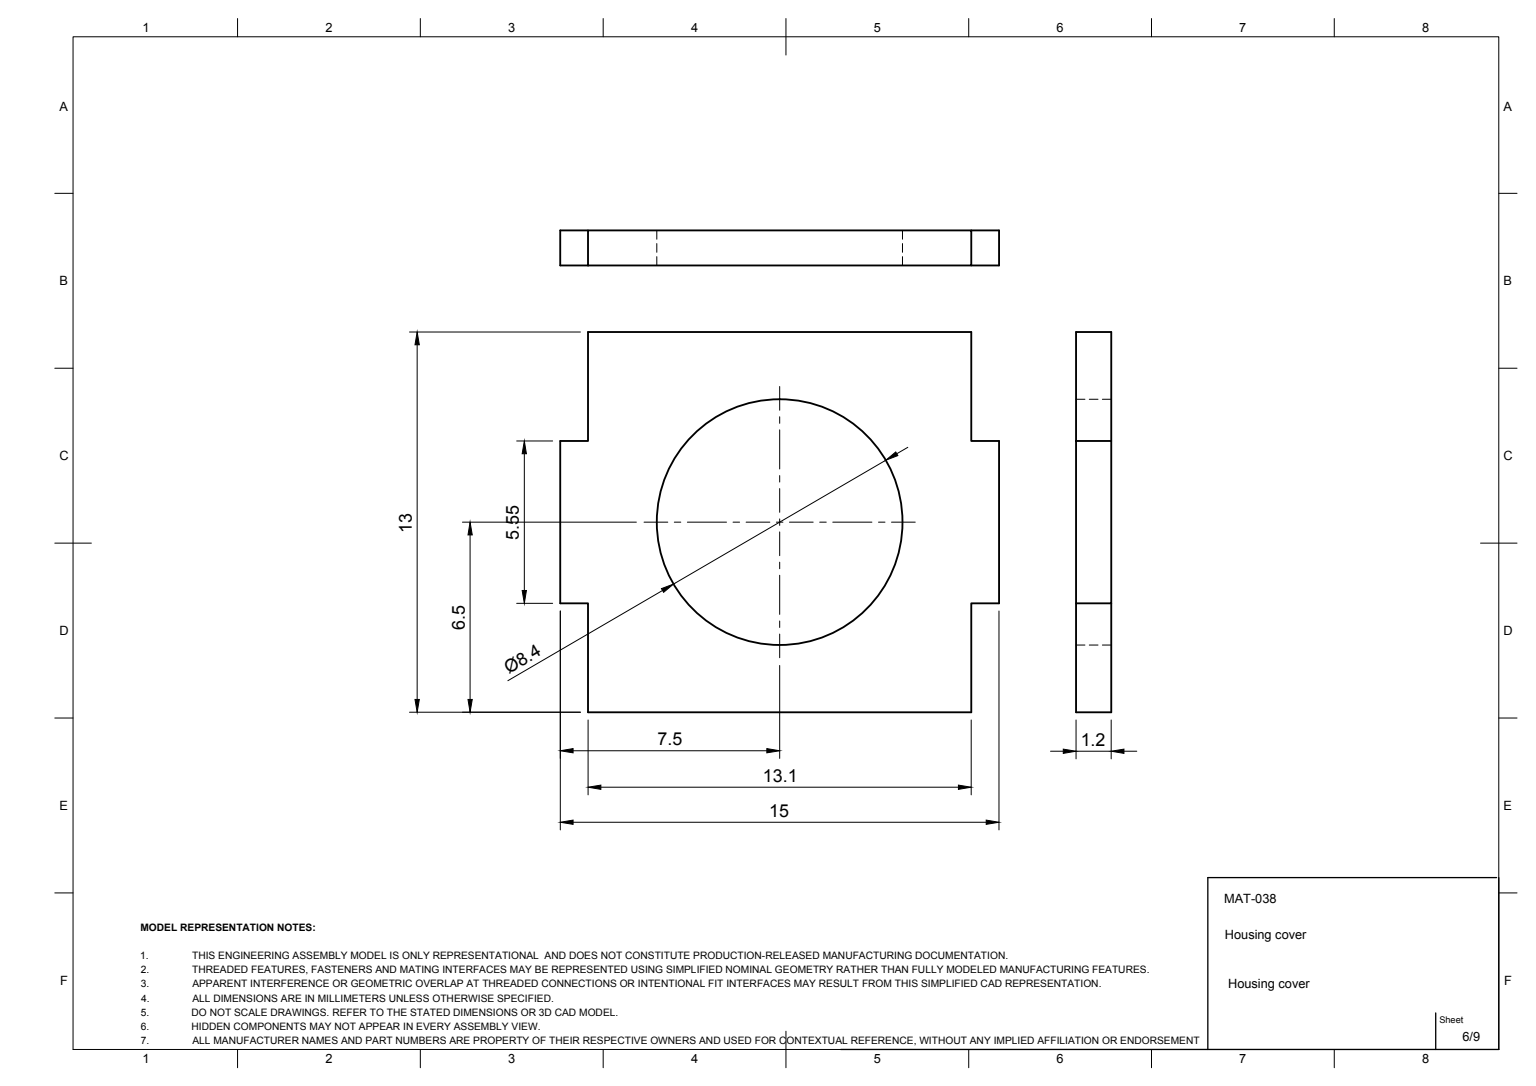
ISO-10303-21;
HEADER;
/* Generated by software containing ST-Developer
 * from STEP Tools, Inc. (www.steptools.com) 
 */

FILE_DESCRIPTION(
/* description */ ('STEP AP214'),
/* implementation_level */ '2;1');

FILE_NAME(
/* name */ 'Housing Cover.step',
/* time_stamp */ '2026-11-14T21:32:33-08:00',
/* author */ (''),
/* organization */ (''),
/* preprocessor_version */ 'ST-DEVELOPER v20.2',
/* originating_system */ 'Autodesk Translation Framework v15.17.0.0',
/* authorisation */ '');

FILE_SCHEMA (('AUTOMOTIVE_DESIGN { 1 0 10303 214 3 1 1 }'));
ENDSEC;

DATA;
#10=MECHANICAL_DESIGN_GEOMETRIC_PRESENTATION_REPRESENTATION('',(#180),#10551);
#162=SHAPE_REPRESENTATION_RELATIONSHIP('SRR','None',#10589,#171);
#171=ADVANCED_BREP_SHAPE_REPRESENTATION('',(#190),#10545);
#180=STYLED_ITEM('',(#10640),#190);
#190=MANIFOLD_SOLID_BREP('Body1',#3429);
#210=FACE_BOUND('',#586,.T.);
#211=FACE_BOUND('',#588,.T.);
#257=PLANE('',#3637);
#258=PLANE('',#3638);
#259=PLANE('',#3639);
#260=PLANE('',#3640);
#261=PLANE('',#3641);
#262=PLANE('',#3642);
#263=PLANE('',#3643);
#264=PLANE('',#3644);
#265=PLANE('',#3645);
#266=PLANE('',#3646);
#267=PLANE('',#3647);
#268=PLANE('',#3648);
#269=PLANE('',#3649);
#270=PLANE('',#3650);
#347=FACE_OUTER_BOUND('',#580,.T.);
#348=FACE_OUTER_BOUND('',#581,.T.);
#349=FACE_OUTER_BOUND('',#582,.T.);
#350=FACE_OUTER_BOUND('',#583,.T.);
#351=FACE_OUTER_BOUND('',#584,.T.);
#352=FACE_OUTER_BOUND('',#585,.T.);
#353=FACE_OUTER_BOUND('',#587,.T.);
#354=FACE_OUTER_BOUND('',#589,.T.);
#355=FACE_OUTER_BOUND('',#590,.T.);
#356=FACE_OUTER_BOUND('',#591,.T.);
#357=FACE_OUTER_BOUND('',#592,.T.);
#358=FACE_OUTER_BOUND('',#593,.T.);
#359=FACE_OUTER_BOUND('',#594,.T.);
#360=FACE_OUTER_BOUND('',#595,.T.);
#361=FACE_OUTER_BOUND('',#596,.T.);
#580=EDGE_LOOP('',(#2452,#2453,#2454,#2455));
#581=EDGE_LOOP('',(#2456,#2457,#2458,#2459));
#582=EDGE_LOOP('',(#2460,#2461,#2462,#2463));
#583=EDGE_LOOP('',(#2464,#2465,#2466,#2467));
#584=EDGE_LOOP('',(#2468,#2469,#2470,#2471));
#585=EDGE_LOOP('',(#2472,#2473,#2474,#2475,#2476,#2477,#2478,#2479,#2480,
#2481,#2482,#2483));
#586=EDGE_LOOP('',(#2484));
#587=EDGE_LOOP('',(#2485,#2486,#2487,#2488,#2489,#2490,#2491,#2492,#2493,
#2494,#2495,#2496));
#588=EDGE_LOOP('',(#2497));
#589=EDGE_LOOP('',(#2498,#2499,#2500,#2501));
#590=EDGE_LOOP('',(#2502,#2503,#2504,#2505));
#591=EDGE_LOOP('',(#2506,#2507,#2508,#2509));
#592=EDGE_LOOP('',(#2510,#2511,#2512,#2513));
#593=EDGE_LOOP('',(#2514,#2515,#2516,#2517));
#594=EDGE_LOOP('',(#2518,#2519,#2520,#2521));
#595=EDGE_LOOP('',(#2522,#2523,#2524,#2525));
#596=EDGE_LOOP('',(#2526,#2527,#2528,#2529));
#853=LINE('',#5515,#1050);
#854=LINE('',#5520,#1051);
#855=LINE('',#5522,#1052);
#856=LINE('',#5524,#1053);
#857=LINE('',#5525,#1054);
#858=LINE('',#5529,#1055);
#859=LINE('',#5531,#1056);
#860=LINE('',#5533,#1057);
#861=LINE('',#5534,#1058);
#862=LINE('',#5538,#1059);
#863=LINE('',#5540,#1060);
#864=LINE('',#5542,#1061);
#865=LINE('',#5543,#1062);
#866=LINE('',#5547,#1063);
#867=LINE('',#5549,#1064);
#868=LINE('',#5551,#1065);
#869=LINE('',#5552,#1066);
#870=LINE('',#5555,#1067);
#871=LINE('',#5556,#1068);
#872=LINE('',#5558,#1069);
#873=LINE('',#5559,#1070);
#874=LINE('',#5561,#1071);
#875=LINE('',#5562,#1072);
#876=LINE('',#5564,#1073);
#877=LINE('',#5565,#1074);
#878=LINE('',#5568,#1075);
#879=LINE('',#5569,#1076);
#880=LINE('',#5571,#1077);
#881=LINE('',#5572,#1078);
#882=LINE('',#5574,#1079);
#883=LINE('',#5575,#1080);
#884=LINE('',#5577,#1081);
#885=LINE('',#5578,#1082);
#886=LINE('',#5580,#1083);
#887=LINE('',#5583,#1084);
#888=LINE('',#5586,#1085);
#889=LINE('',#5589,#1086);
#1050=VECTOR('',#4328,4.2);
#1051=VECTOR('',#4333,1000.);
#1052=VECTOR('',#4334,1000.);
#1053=VECTOR('',#4335,1000.);
#1054=VECTOR('',#4336,1000.);
#1055=VECTOR('',#4339,1000.);
#1056=VECTOR('',#4340,1000.);
#1057=VECTOR('',#4341,1000.);
#1058=VECTOR('',#4342,1000.);
#1059=VECTOR('',#4345,1000.);
#1060=VECTOR('',#4346,1000.);
#1061=VECTOR('',#4347,1000.);
#1062=VECTOR('',#4348,1000.);
#1063=VECTOR('',#4351,1000.);
#1064=VECTOR('',#4352,1000.);
#1065=VECTOR('',#4353,1000.);
#1066=VECTOR('',#4354,1000.);
#1067=VECTOR('',#4357,1000.);
#1068=VECTOR('',#4358,1000.);
#1069=VECTOR('',#4359,1000.);
#1070=VECTOR('',#4360,1000.);
#1071=VECTOR('',#4361,1000.);
#1072=VECTOR('',#4362,1000.);
#1073=VECTOR('',#4363,1000.);
#1074=VECTOR('',#4364,1000.);
#1075=VECTOR('',#4367,1000.);
#1076=VECTOR('',#4368,1000.);
#1077=VECTOR('',#4369,1000.);
#1078=VECTOR('',#4370,1000.);
#1079=VECTOR('',#4371,1000.);
#1080=VECTOR('',#4372,1000.);
#1081=VECTOR('',#4373,1000.);
#1082=VECTOR('',#4374,1000.);
#1083=VECTOR('',#4377,1000.);
#1084=VECTOR('',#4382,1000.);
#1085=VECTOR('',#4387,1000.);
#1086=VECTOR('',#4392,1000.);
#1195=CIRCLE('',#3635,4.2);
#1196=CIRCLE('',#3636,4.2);
#1509=VERTEX_POINT('',#5512);
#1510=VERTEX_POINT('',#5514);
#1511=VERTEX_POINT('',#5518);
#1512=VERTEX_POINT('',#5519);
#1513=VERTEX_POINT('',#5521);
#1514=VERTEX_POINT('',#5523);
#1515=VERTEX_POINT('',#5527);
#1516=VERTEX_POINT('',#5528);
#1517=VERTEX_POINT('',#5530);
#1518=VERTEX_POINT('',#5532);
#1519=VERTEX_POINT('',#5536);
#1520=VERTEX_POINT('',#5537);
#1521=VERTEX_POINT('',#5539);
#1522=VERTEX_POINT('',#5541);
#1523=VERTEX_POINT('',#5545);
#1524=VERTEX_POINT('',#5546);
#1525=VERTEX_POINT('',#5548);
#1526=VERTEX_POINT('',#5550);
#1527=VERTEX_POINT('',#5554);
#1528=VERTEX_POINT('',#5557);
#1529=VERTEX_POINT('',#5560);
#1530=VERTEX_POINT('',#5563);
#1531=VERTEX_POINT('',#5567);
#1532=VERTEX_POINT('',#5570);
#1533=VERTEX_POINT('',#5573);
#1534=VERTEX_POINT('',#5576);
#1839=EDGE_CURVE('',#1509,#1509,#1195,.T.);
#1840=EDGE_CURVE('',#1509,#1510,#853,.T.);
#1841=EDGE_CURVE('',#1510,#1510,#1196,.T.);
#1842=EDGE_CURVE('',#1511,#1512,#854,.T.);
#1843=EDGE_CURVE('',#1513,#1511,#855,.T.);
#1844=EDGE_CURVE('',#1513,#1514,#856,.T.);
#1845=EDGE_CURVE('',#1514,#1512,#857,.T.);
#1846=EDGE_CURVE('',#1515,#1516,#858,.T.);
#1847=EDGE_CURVE('',#1517,#1515,#859,.T.);
#1848=EDGE_CURVE('',#1517,#1518,#860,.T.);
#1849=EDGE_CURVE('',#1518,#1516,#861,.T.);
#1850=EDGE_CURVE('',#1519,#1520,#862,.T.);
#1851=EDGE_CURVE('',#1521,#1519,#863,.T.);
#1852=EDGE_CURVE('',#1521,#1522,#864,.T.);
#1853=EDGE_CURVE('',#1522,#1520,#865,.T.);
#1854=EDGE_CURVE('',#1523,#1524,#866,.T.);
#1855=EDGE_CURVE('',#1524,#1525,#867,.T.);
#1856=EDGE_CURVE('',#1526,#1525,#868,.T.);
#1857=EDGE_CURVE('',#1523,#1526,#869,.T.);
#1858=EDGE_CURVE('',#1527,#1525,#870,.T.);
#1859=EDGE_CURVE('',#1511,#1527,#871,.T.);
#1860=EDGE_CURVE('',#1528,#1512,#872,.T.);
#1861=EDGE_CURVE('',#1515,#1528,#873,.T.);
#1862=EDGE_CURVE('',#1529,#1516,#874,.T.);
#1863=EDGE_CURVE('',#1519,#1529,#875,.T.);
#1864=EDGE_CURVE('',#1530,#1520,#876,.T.);
#1865=EDGE_CURVE('',#1526,#1530,#877,.T.);
#1866=EDGE_CURVE('',#1531,#1513,#878,.T.);
#1867=EDGE_CURVE('',#1524,#1531,#879,.T.);
#1868=EDGE_CURVE('',#1532,#1523,#880,.T.);
#1869=EDGE_CURVE('',#1522,#1532,#881,.T.);
#1870=EDGE_CURVE('',#1533,#1521,#882,.T.);
#1871=EDGE_CURVE('',#1518,#1533,#883,.T.);
#1872=EDGE_CURVE('',#1534,#1517,#884,.T.);
#1873=EDGE_CURVE('',#1514,#1534,#885,.T.);
#1874=EDGE_CURVE('',#1532,#1530,#886,.T.);
#1875=EDGE_CURVE('',#1533,#1529,#887,.T.);
#1876=EDGE_CURVE('',#1534,#1528,#888,.T.);
#1877=EDGE_CURVE('',#1531,#1527,#889,.T.);
#2452=ORIENTED_EDGE('',*,*,#1839,.T.);
#2453=ORIENTED_EDGE('',*,*,#1840,.T.);
#2454=ORIENTED_EDGE('',*,*,#1841,.T.);
#2455=ORIENTED_EDGE('',*,*,#1840,.F.);
#2456=ORIENTED_EDGE('',*,*,#1842,.F.);
#2457=ORIENTED_EDGE('',*,*,#1843,.F.);
#2458=ORIENTED_EDGE('',*,*,#1844,.T.);
#2459=ORIENTED_EDGE('',*,*,#1845,.T.);
#2460=ORIENTED_EDGE('',*,*,#1846,.F.);
#2461=ORIENTED_EDGE('',*,*,#1847,.F.);
#2462=ORIENTED_EDGE('',*,*,#1848,.T.);
#2463=ORIENTED_EDGE('',*,*,#1849,.T.);
#2464=ORIENTED_EDGE('',*,*,#1850,.F.);
#2465=ORIENTED_EDGE('',*,*,#1851,.F.);
#2466=ORIENTED_EDGE('',*,*,#1852,.T.);
#2467=ORIENTED_EDGE('',*,*,#1853,.T.);
#2468=ORIENTED_EDGE('',*,*,#1854,.T.);
#2469=ORIENTED_EDGE('',*,*,#1855,.T.);
#2470=ORIENTED_EDGE('',*,*,#1856,.F.);
#2471=ORIENTED_EDGE('',*,*,#1857,.F.);
#2472=ORIENTED_EDGE('',*,*,#1858,.F.);
#2473=ORIENTED_EDGE('',*,*,#1859,.F.);
#2474=ORIENTED_EDGE('',*,*,#1842,.T.);
#2475=ORIENTED_EDGE('',*,*,#1860,.F.);
#2476=ORIENTED_EDGE('',*,*,#1861,.F.);
#2477=ORIENTED_EDGE('',*,*,#1846,.T.);
#2478=ORIENTED_EDGE('',*,*,#1862,.F.);
#2479=ORIENTED_EDGE('',*,*,#1863,.F.);
#2480=ORIENTED_EDGE('',*,*,#1850,.T.);
#2481=ORIENTED_EDGE('',*,*,#1864,.F.);
#2482=ORIENTED_EDGE('',*,*,#1865,.F.);
#2483=ORIENTED_EDGE('',*,*,#1856,.T.);
#2484=ORIENTED_EDGE('',*,*,#1841,.F.);
#2485=ORIENTED_EDGE('',*,*,#1866,.F.);
#2486=ORIENTED_EDGE('',*,*,#1867,.F.);
#2487=ORIENTED_EDGE('',*,*,#1854,.F.);
#2488=ORIENTED_EDGE('',*,*,#1868,.F.);
#2489=ORIENTED_EDGE('',*,*,#1869,.F.);
#2490=ORIENTED_EDGE('',*,*,#1852,.F.);
#2491=ORIENTED_EDGE('',*,*,#1870,.F.);
#2492=ORIENTED_EDGE('',*,*,#1871,.F.);
#2493=ORIENTED_EDGE('',*,*,#1848,.F.);
#2494=ORIENTED_EDGE('',*,*,#1872,.F.);
#2495=ORIENTED_EDGE('',*,*,#1873,.F.);
#2496=ORIENTED_EDGE('',*,*,#1844,.F.);
#2497=ORIENTED_EDGE('',*,*,#1839,.F.);
#2498=ORIENTED_EDGE('',*,*,#1869,.T.);
#2499=ORIENTED_EDGE('',*,*,#1874,.T.);
#2500=ORIENTED_EDGE('',*,*,#1864,.T.);
#2501=ORIENTED_EDGE('',*,*,#1853,.F.);
#2502=ORIENTED_EDGE('',*,*,#1868,.T.);
#2503=ORIENTED_EDGE('',*,*,#1857,.T.);
#2504=ORIENTED_EDGE('',*,*,#1865,.T.);
#2505=ORIENTED_EDGE('',*,*,#1874,.F.);
#2506=ORIENTED_EDGE('',*,*,#1871,.T.);
#2507=ORIENTED_EDGE('',*,*,#1875,.T.);
#2508=ORIENTED_EDGE('',*,*,#1862,.T.);
#2509=ORIENTED_EDGE('',*,*,#1849,.F.);
#2510=ORIENTED_EDGE('',*,*,#1870,.T.);
#2511=ORIENTED_EDGE('',*,*,#1851,.T.);
#2512=ORIENTED_EDGE('',*,*,#1863,.T.);
#2513=ORIENTED_EDGE('',*,*,#1875,.F.);
#2514=ORIENTED_EDGE('',*,*,#1873,.T.);
#2515=ORIENTED_EDGE('',*,*,#1876,.T.);
#2516=ORIENTED_EDGE('',*,*,#1860,.T.);
#2517=ORIENTED_EDGE('',*,*,#1845,.F.);
#2518=ORIENTED_EDGE('',*,*,#1872,.T.);
#2519=ORIENTED_EDGE('',*,*,#1847,.T.);
#2520=ORIENTED_EDGE('',*,*,#1861,.T.);
#2521=ORIENTED_EDGE('',*,*,#1876,.F.);
#2522=ORIENTED_EDGE('',*,*,#1867,.T.);
#2523=ORIENTED_EDGE('',*,*,#1877,.T.);
#2524=ORIENTED_EDGE('',*,*,#1858,.T.);
#2525=ORIENTED_EDGE('',*,*,#1855,.F.);
#2526=ORIENTED_EDGE('',*,*,#1866,.T.);
#2527=ORIENTED_EDGE('',*,*,#1843,.T.);
#2528=ORIENTED_EDGE('',*,*,#1859,.T.);
#2529=ORIENTED_EDGE('',*,*,#1877,.F.);
#3170=CYLINDRICAL_SURFACE('',#3634,4.2);
#3259=ADVANCED_FACE('',(#347),#3170,.F.);
#3260=ADVANCED_FACE('',(#348),#257,.F.);
#3261=ADVANCED_FACE('',(#349),#258,.F.);
#3262=ADVANCED_FACE('',(#350),#259,.F.);
#3263=ADVANCED_FACE('',(#351),#260,.F.);
#3264=ADVANCED_FACE('',(#352,#210),#261,.T.);
#3265=ADVANCED_FACE('',(#353,#211),#262,.F.);
#3266=ADVANCED_FACE('',(#354),#263,.F.);
#3267=ADVANCED_FACE('',(#355),#264,.F.);
#3268=ADVANCED_FACE('',(#356),#265,.F.);
#3269=ADVANCED_FACE('',(#357),#266,.F.);
#3270=ADVANCED_FACE('',(#358),#267,.F.);
#3271=ADVANCED_FACE('',(#359),#268,.F.);
#3272=ADVANCED_FACE('',(#360),#269,.F.);
#3273=ADVANCED_FACE('',(#361),#270,.F.);
#3429=CLOSED_SHELL('',(#3259,#3260,#3261,#3262,#3263,#3264,#3265,#3266,
#3267,#3268,#3269,#3270,#3271,#3272,#3273));
#3633=AXIS2_PLACEMENT_3D('',#5510,#4322,#4323);
#3634=AXIS2_PLACEMENT_3D('',#5511,#4324,#4325);
#3635=AXIS2_PLACEMENT_3D('',#5513,#4326,#4327);
#3636=AXIS2_PLACEMENT_3D('',#5516,#4329,#4330);
#3637=AXIS2_PLACEMENT_3D('',#5517,#4331,#4332);
#3638=AXIS2_PLACEMENT_3D('',#5526,#4337,#4338);
#3639=AXIS2_PLACEMENT_3D('',#5535,#4343,#4344);
#3640=AXIS2_PLACEMENT_3D('',#5544,#4349,#4350);
#3641=AXIS2_PLACEMENT_3D('',#5553,#4355,#4356);
#3642=AXIS2_PLACEMENT_3D('',#5566,#4365,#4366);
#3643=AXIS2_PLACEMENT_3D('',#5579,#4375,#4376);
#3644=AXIS2_PLACEMENT_3D('',#5581,#4378,#4379);
#3645=AXIS2_PLACEMENT_3D('',#5582,#4380,#4381);
#3646=AXIS2_PLACEMENT_3D('',#5584,#4383,#4384);
#3647=AXIS2_PLACEMENT_3D('',#5585,#4385,#4386);
#3648=AXIS2_PLACEMENT_3D('',#5587,#4388,#4389);
#3649=AXIS2_PLACEMENT_3D('',#5588,#4390,#4391);
#3650=AXIS2_PLACEMENT_3D('',#5590,#4393,#4394);
#4322=DIRECTION('axis',(0.,0.,1.));
#4323=DIRECTION('refdir',(1.,0.,0.));
#4324=DIRECTION('center_axis',(0.,0.,1.));
#4325=DIRECTION('ref_axis',(1.,0.,0.));
#4326=DIRECTION('center_axis',(0.,0.,-1.));
#4327=DIRECTION('ref_axis',(1.,0.,0.));
#4328=DIRECTION('',(0.,0.,1.));
#4329=DIRECTION('center_axis',(0.,0.,1.));
#4330=DIRECTION('ref_axis',(1.,0.,0.));
#4331=DIRECTION('center_axis',(1.,1.33440267382831E-16,0.));
#4332=DIRECTION('ref_axis',(-1.33440267382831E-16,1.,0.));
#4333=DIRECTION('',(1.33440267382831E-16,-1.,0.));
#4334=DIRECTION('',(0.,0.,1.));
#4335=DIRECTION('',(1.33440267382831E-16,-1.,0.));
#4336=DIRECTION('',(0.,0.,1.));
#4337=DIRECTION('center_axis',(0.,1.,0.));
#4338=DIRECTION('ref_axis',(0.,0.,1.));
#4339=DIRECTION('',(1.,0.,0.));
#4340=DIRECTION('',(0.,0.,1.));
#4341=DIRECTION('',(1.,0.,0.));
#4342=DIRECTION('',(0.,0.,1.));
#4343=DIRECTION('center_axis',(-1.,0.,0.));
#4344=DIRECTION('ref_axis',(0.,0.,1.));
#4345=DIRECTION('',(0.,1.,0.));
#4346=DIRECTION('',(0.,0.,1.));
#4347=DIRECTION('',(0.,1.,0.));
#4348=DIRECTION('',(0.,0.,1.));
#4349=DIRECTION('center_axis',(0.,-1.,0.));
#4350=DIRECTION('ref_axis',(0.,0.,-1.));
#4351=DIRECTION('',(-1.,0.,0.));
#4352=DIRECTION('',(0.,0.,1.));
#4353=DIRECTION('',(-1.,0.,0.));
#4354=DIRECTION('',(0.,0.,1.));
#4355=DIRECTION('center_axis',(0.,0.,1.));
#4356=DIRECTION('ref_axis',(1.,0.,0.));
#4357=DIRECTION('',(2.32848788721719E-16,1.,0.));
#4358=DIRECTION('',(1.,0.,0.));
#4359=DIRECTION('',(-1.,0.,0.));
#4360=DIRECTION('',(-2.32848788721719E-16,1.,0.));
#4361=DIRECTION('',(0.,-1.,0.));
#4362=DIRECTION('',(-1.,0.,0.));
#4363=DIRECTION('',(1.,0.,0.));
#4364=DIRECTION('',(0.,-1.,0.));
#4365=DIRECTION('center_axis',(0.,0.,1.));
#4366=DIRECTION('ref_axis',(1.,0.,0.));
#4367=DIRECTION('',(-1.,0.,0.));
#4368=DIRECTION('',(-2.32848788721719E-16,-1.,0.));
#4369=DIRECTION('',(0.,1.,0.));
#4370=DIRECTION('',(-1.,0.,0.));
#4371=DIRECTION('',(1.,0.,0.));
#4372=DIRECTION('',(0.,1.,0.));
#4373=DIRECTION('',(2.32848788721719E-16,-1.,0.));
#4374=DIRECTION('',(1.,0.,0.));
#4375=DIRECTION('center_axis',(0.,-1.,0.));
#4376=DIRECTION('ref_axis',(0.,0.,-1.));
#4377=DIRECTION('',(0.,0.,1.));
#4378=DIRECTION('center_axis',(-1.,0.,0.));
#4379=DIRECTION('ref_axis',(0.,0.,1.));
#4380=DIRECTION('center_axis',(-1.,0.,0.));
#4381=DIRECTION('ref_axis',(0.,0.,1.));
#4382=DIRECTION('',(0.,0.,1.));
#4383=DIRECTION('center_axis',(0.,1.,0.));
#4384=DIRECTION('ref_axis',(0.,0.,1.));
#4385=DIRECTION('center_axis',(0.,1.,0.));
#4386=DIRECTION('ref_axis',(0.,0.,1.));
#4387=DIRECTION('',(0.,0.,1.));
#4388=DIRECTION('center_axis',(1.,2.32848788721719E-16,0.));
#4389=DIRECTION('ref_axis',(-2.32848788721719E-16,1.,0.));
#4390=DIRECTION('center_axis',(1.,-2.32848788721719E-16,0.));
#4391=DIRECTION('ref_axis',(2.32848788721719E-16,1.,0.));
#4392=DIRECTION('',(0.,0.,1.));
#4393=DIRECTION('center_axis',(0.,-1.,0.));
#4394=DIRECTION('ref_axis',(0.,0.,-1.));
#5510=CARTESIAN_POINT('',(0.,0.,0.));
#5511=CARTESIAN_POINT('Origin',(0.,0.,-0.000999999999999916));
#5512=CARTESIAN_POINT('',(-4.2,-5.14351655641888E-16,0.));
#5513=CARTESIAN_POINT('Origin',(0.,0.,0.));
#5514=CARTESIAN_POINT('',(-4.2,-5.14351655641888E-16,1.2));
#5515=CARTESIAN_POINT('',(-4.2,-5.14351655641888E-16,-0.000999999999999916));
#5516=CARTESIAN_POINT('Origin',(0.,0.,1.2));
#5517=CARTESIAN_POINT('Origin',(-7.5,6.5,1.2));
#5518=CARTESIAN_POINT('',(-7.5,2.775,1.2));
#5519=CARTESIAN_POINT('',(-7.5,-2.775,1.2));
#5520=CARTESIAN_POINT('',(-7.5,6.5,1.2));
#5521=CARTESIAN_POINT('',(-7.5,2.775,0.));
#5522=CARTESIAN_POINT('',(-7.5,2.775,-0.000999999999999916));
#5523=CARTESIAN_POINT('',(-7.5,-2.775,0.));
#5524=CARTESIAN_POINT('',(-7.5,6.5,0.));
#5525=CARTESIAN_POINT('',(-7.5,-2.775,-0.000999999999999916));
#5526=CARTESIAN_POINT('Origin',(-7.5,-6.5,1.2));
#5527=CARTESIAN_POINT('',(-6.55,-6.5,1.2));
#5528=CARTESIAN_POINT('',(6.55,-6.5,1.2));
#5529=CARTESIAN_POINT('',(-7.5,-6.5,1.2));
#5530=CARTESIAN_POINT('',(-6.55,-6.5,0.));
#5531=CARTESIAN_POINT('',(-6.55,-6.5,-0.000999999999999916));
#5532=CARTESIAN_POINT('',(6.55,-6.5,0.));
#5533=CARTESIAN_POINT('',(-7.5,-6.5,0.));
#5534=CARTESIAN_POINT('',(6.55,-6.5,-0.000999999999999916));
#5535=CARTESIAN_POINT('Origin',(7.5,6.5,1.2));
#5536=CARTESIAN_POINT('',(7.5,-2.775,1.2));
#5537=CARTESIAN_POINT('',(7.5,2.775,1.2));
#5538=CARTESIAN_POINT('',(7.5,6.5,1.2));
#5539=CARTESIAN_POINT('',(7.5,-2.775,0.));
#5540=CARTESIAN_POINT('',(7.5,-2.775,-0.000999999999999916));
#5541=CARTESIAN_POINT('',(7.5,2.775,0.));
#5542=CARTESIAN_POINT('',(7.5,6.5,0.));
#5543=CARTESIAN_POINT('',(7.5,2.775,-0.000999999999999916));
#5544=CARTESIAN_POINT('Origin',(-7.5,6.5,1.2));
#5545=CARTESIAN_POINT('',(6.55,6.5,0.));
#5546=CARTESIAN_POINT('',(-6.55,6.5,0.));
#5547=CARTESIAN_POINT('',(-7.5,6.5,0.));
#5548=CARTESIAN_POINT('',(-6.55,6.5,1.2));
#5549=CARTESIAN_POINT('',(-6.55,6.5,-0.000999999999999916));
#5550=CARTESIAN_POINT('',(6.55,6.5,1.2));
#5551=CARTESIAN_POINT('',(-7.5,6.5,1.2));
#5552=CARTESIAN_POINT('',(6.55,6.5,-0.000999999999999916));
#5553=CARTESIAN_POINT('Origin',(0.,0.,1.2));
#5554=CARTESIAN_POINT('',(-6.55,2.775,1.2));
#5555=CARTESIAN_POINT('',(-6.55,6.5,1.2));
#5556=CARTESIAN_POINT('',(-7.5,2.775,1.2));
#5557=CARTESIAN_POINT('',(-6.55,-2.775,1.2));
#5558=CARTESIAN_POINT('',(-7.5,-2.775,1.2));
#5559=CARTESIAN_POINT('',(-6.55,-6.5,1.2));
#5560=CARTESIAN_POINT('',(6.55,-2.775,1.2));
#5561=CARTESIAN_POINT('',(6.55,-6.5,1.2));
#5562=CARTESIAN_POINT('',(7.5,-2.775,1.2));
#5563=CARTESIAN_POINT('',(6.55,2.775,1.2));
#5564=CARTESIAN_POINT('',(7.5,2.775,1.2));
#5565=CARTESIAN_POINT('',(6.55,6.5,1.2));
#5566=CARTESIAN_POINT('Origin',(0.,0.,0.));
#5567=CARTESIAN_POINT('',(-6.55,2.775,0.));
#5568=CARTESIAN_POINT('',(-7.5,2.775,0.));
#5569=CARTESIAN_POINT('',(-6.55,6.5,0.));
#5570=CARTESIAN_POINT('',(6.55,2.775,0.));
#5571=CARTESIAN_POINT('',(6.55,6.5,0.));
#5572=CARTESIAN_POINT('',(7.5,2.775,0.));
#5573=CARTESIAN_POINT('',(6.55,-2.775,0.));
#5574=CARTESIAN_POINT('',(7.5,-2.775,0.));
#5575=CARTESIAN_POINT('',(6.55,-6.5,0.));
#5576=CARTESIAN_POINT('',(-6.55,-2.775,0.));
#5577=CARTESIAN_POINT('',(-6.55,-6.5,0.));
#5578=CARTESIAN_POINT('',(-7.5,-2.775,0.));
#5579=CARTESIAN_POINT('Origin',(7.5,2.775,-0.000999999999999916));
#5580=CARTESIAN_POINT('',(6.55,2.775,-0.000999999999999916));
#5581=CARTESIAN_POINT('Origin',(6.55,6.5,-0.000999999999999916));
#5582=CARTESIAN_POINT('Origin',(6.55,-6.5,-0.000999999999999916));
#5583=CARTESIAN_POINT('',(6.55,-2.775,-0.000999999999999916));
#5584=CARTESIAN_POINT('Origin',(7.5,-2.775,-0.000999999999999916));
#5585=CARTESIAN_POINT('Origin',(-7.5,-2.775,-0.000999999999999916));
#5586=CARTESIAN_POINT('',(-6.55,-2.775,-0.000999999999999916));
#5587=CARTESIAN_POINT('Origin',(-6.55,-6.5,-0.000999999999999916));
#5588=CARTESIAN_POINT('Origin',(-6.55,6.5,-0.000999999999999916));
#5589=CARTESIAN_POINT('',(-6.55,2.775,-0.000999999999999916));
#5590=CARTESIAN_POINT('Origin',(-7.5,2.775,-0.000999999999999916));
#10534=UNCERTAINTY_MEASURE_WITH_UNIT(LENGTH_MEASURE(0.01),#10552,
'DISTANCE_ACCURACY_VALUE',
'Maximum model space distance between geometric entities at asserted c
onnectivities');
#10540=UNCERTAINTY_MEASURE_WITH_UNIT(LENGTH_MEASURE(0.01),#10552,
'DISTANCE_ACCURACY_VALUE',
'Maximum model space distance between geometric entities at asserted c
onnectivities');
#10545=(
GEOMETRIC_REPRESENTATION_CONTEXT(3)
GLOBAL_UNCERTAINTY_ASSIGNED_CONTEXT((#10534))
GLOBAL_UNIT_ASSIGNED_CONTEXT((#10552,#10554,#10555))
REPRESENTATION_CONTEXT('','3D')
);
#10551=(
GEOMETRIC_REPRESENTATION_CONTEXT(3)
GLOBAL_UNCERTAINTY_ASSIGNED_CONTEXT((#10540))
GLOBAL_UNIT_ASSIGNED_CONTEXT((#10552,#10554,#10555))
REPRESENTATION_CONTEXT('','3D')
);
#10552=(
LENGTH_UNIT()
NAMED_UNIT(*)
SI_UNIT(.MILLI.,.METRE.)
);
#10554=(
NAMED_UNIT(*)
PLANE_ANGLE_UNIT()
SI_UNIT($,.RADIAN.)
);
#10555=(
NAMED_UNIT(*)
SI_UNIT($,.STERADIAN.)
SOLID_ANGLE_UNIT()
);
#10560=SHAPE_DEFINITION_REPRESENTATION(#10570,#10589);
#10570=PRODUCT_DEFINITION_SHAPE('',$,#10600);
#10589=SHAPE_REPRESENTATION('',(#3633),#10545);
#10595=PRODUCT_DEFINITION_CONTEXT('part definition',#10627,'design');
#10600=PRODUCT_DEFINITION('Housing cover','Housing Cover',#10610,#10595);
#10610=PRODUCT_DEFINITION_FORMATION('',$,#10633);
#10627=APPLICATION_CONTEXT(
'Core Data for Automotive Mechanical Design Process');
#10628=PRODUCT_CONTEXT('part definition',#10627,'mechanical');
#10633=PRODUCT('Housing cover','Housing Cover',$,(#10628));
#10640=PRESENTATION_STYLE_ASSIGNMENT((#10647));
#10647=SURFACE_STYLE_USAGE(.BOTH.,#10654);
#10654=SURFACE_SIDE_STYLE('',(#10661));
#10661=SURFACE_STYLE_FILL_AREA(#10668);
#10668=FILL_AREA_STYLE('Opaque(20,51,87)',(#10675));
#10675=FILL_AREA_STYLE_COLOUR('Opaque(20,51,87)',#10682);
#10682=COLOUR_RGB('Opaque(20,51,87)',0.0784313725490196,0.2,0.341176470588235);
ENDSEC;
END-ISO-10303-21;
